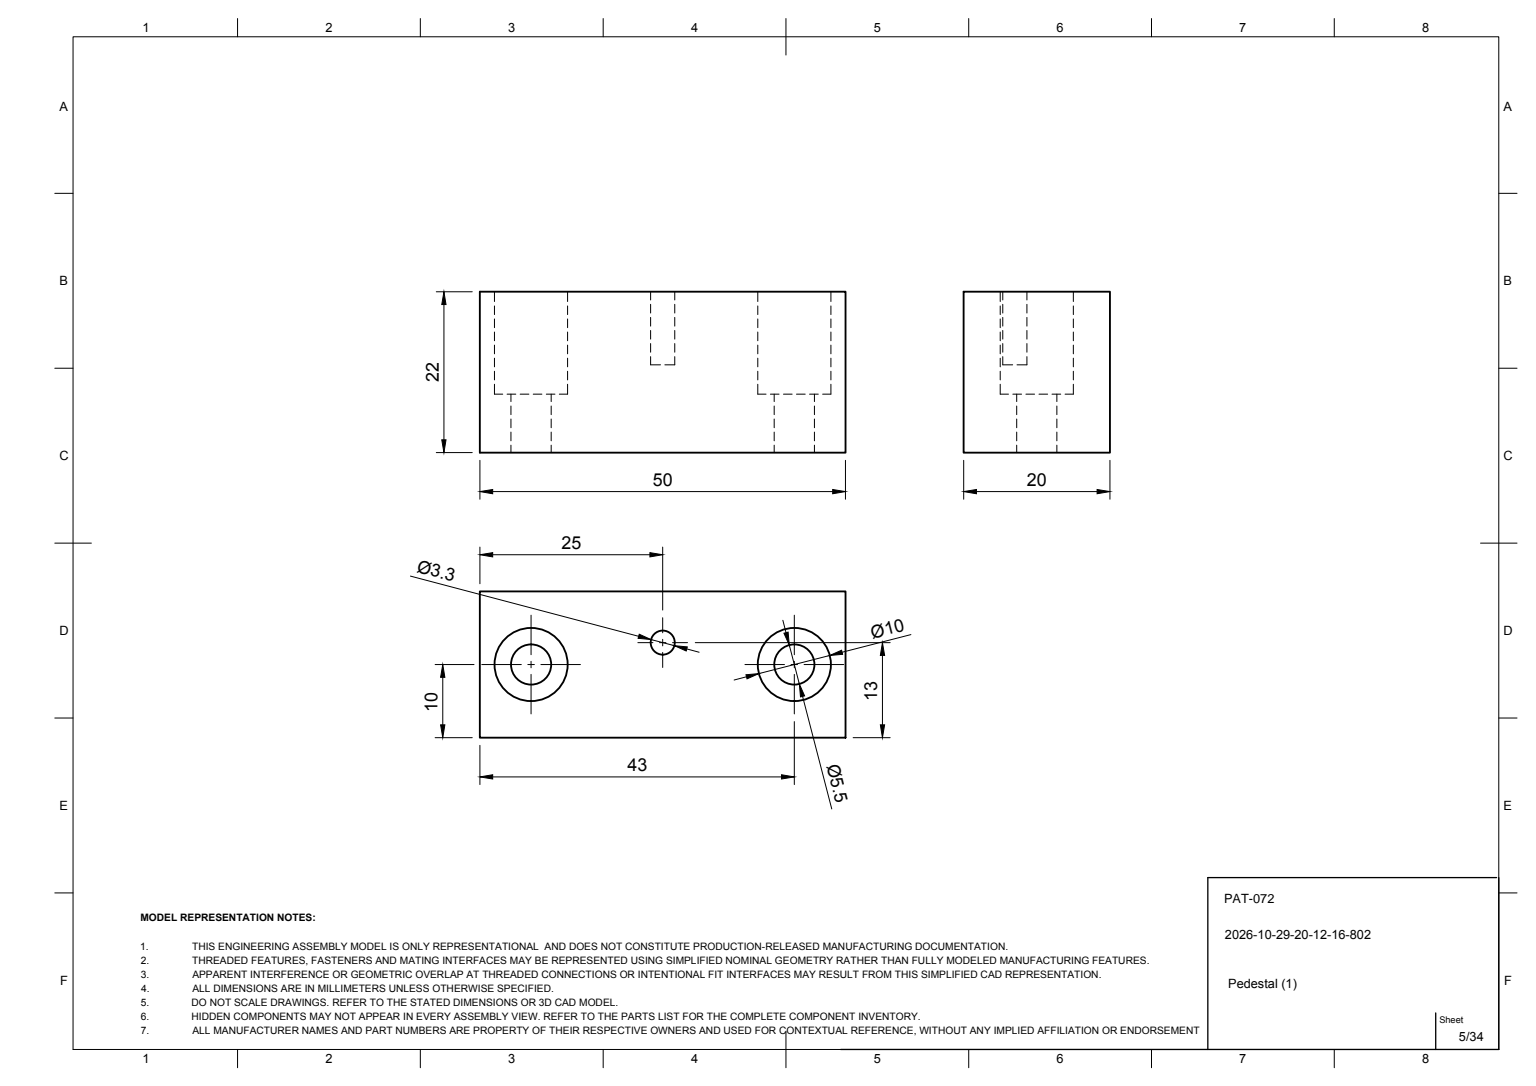
ISO-10303-21;
HEADER;
/* Generated by software containing ST-Developer
 * from STEP Tools, Inc. (www.steptools.com) 
 */

FILE_DESCRIPTION(
/* description */ ('PAT-072'),
/* implementation_level */ '2;1');

FILE_NAME(
/* name */ 'Pedestal (1).step',
/* time_stamp */ '2026-10-29T20:11:56-07:00',
/* author */ (''),
/* organization */ (''),
/* preprocessor_version */ 'ST-DEVELOPER v20.2',
/* originating_system */ 'Autodesk Translation Framework v15.17.0.0',
/* authorisation */ '');

FILE_SCHEMA (('AUTOMOTIVE_DESIGN { 1 0 10303 214 3 1 1 }'));
ENDSEC;

DATA;
#10=MECHANICAL_DESIGN_GEOMETRIC_PRESENTATION_REPRESENTATION('',(#334),#11432);
#262=SHAPE_REPRESENTATION_RELATIONSHIP('SRR','None',#11566,#298);
#298=ADVANCED_BREP_SHAPE_REPRESENTATION('',(#370),#11397);
#334=STYLED_ITEM('',(#11805),#370);
#370=MANIFOLD_SOLID_BREP('Body1',#6069);
#417=FACE_BOUND('',#1211,.T.);
#418=FACE_BOUND('',#1214,.T.);
#419=FACE_BOUND('',#1222,.T.);
#420=FACE_BOUND('',#1223,.T.);
#421=FACE_BOUND('',#1224,.T.);
#422=FACE_BOUND('',#1226,.T.);
#423=FACE_BOUND('',#1227,.T.);
#585=PLANE('',#6551);
#586=PLANE('',#6555);
#587=PLANE('',#6560);
#588=PLANE('',#6566);
#589=PLANE('',#6567);
#590=PLANE('',#6568);
#591=PLANE('',#6569);
#592=PLANE('',#6570);
#593=PLANE('',#6571);
#820=FACE_OUTER_BOUND('',#1207,.T.);
#821=FACE_OUTER_BOUND('',#1208,.T.);
#822=FACE_OUTER_BOUND('',#1209,.T.);
#823=FACE_OUTER_BOUND('',#1210,.T.);
#824=FACE_OUTER_BOUND('',#1212,.T.);
#825=FACE_OUTER_BOUND('',#1213,.T.);
#826=FACE_OUTER_BOUND('',#1215,.T.);
#827=FACE_OUTER_BOUND('',#1216,.T.);
#828=FACE_OUTER_BOUND('',#1217,.T.);
#829=FACE_OUTER_BOUND('',#1218,.T.);
#830=FACE_OUTER_BOUND('',#1219,.T.);
#831=FACE_OUTER_BOUND('',#1220,.T.);
#832=FACE_OUTER_BOUND('',#1221,.T.);
#833=FACE_OUTER_BOUND('',#1225,.T.);
#1207=EDGE_LOOP('',(#4170,#4171,#4172,#4173));
#1208=EDGE_LOOP('',(#4174));
#1209=EDGE_LOOP('',(#4175,#4176,#4177,#4178));
#1210=EDGE_LOOP('',(#4179));
#1211=EDGE_LOOP('',(#4180));
#1212=EDGE_LOOP('',(#4181,#4182,#4183,#4184));
#1213=EDGE_LOOP('',(#4185));
#1214=EDGE_LOOP('',(#4186));
#1215=EDGE_LOOP('',(#4187,#4188,#4189,#4190));
#1216=EDGE_LOOP('',(#4191,#4192,#4193,#4194));
#1217=EDGE_LOOP('',(#4195,#4196,#4197,#4198));
#1218=EDGE_LOOP('',(#4199,#4200,#4201,#4202));
#1219=EDGE_LOOP('',(#4203,#4204,#4205,#4206));
#1220=EDGE_LOOP('',(#4207,#4208,#4209,#4210));
#1221=EDGE_LOOP('',(#4211,#4212,#4213,#4214));
#1222=EDGE_LOOP('',(#4215));
#1223=EDGE_LOOP('',(#4216));
#1224=EDGE_LOOP('',(#4217));
#1225=EDGE_LOOP('',(#4218,#4219,#4220,#4221));
#1226=EDGE_LOOP('',(#4222));
#1227=EDGE_LOOP('',(#4223));
#1741=LINE('',#9309,#2160);
#1742=LINE('',#9316,#2161);
#1743=LINE('',#9325,#2162);
#1744=LINE('',#9333,#2163);
#1745=LINE('',#9337,#2164);
#1746=LINE('',#9341,#2165);
#1747=LINE('',#9343,#2166);
#1748=LINE('',#9345,#2167);
#1749=LINE('',#9346,#2168);
#1750=LINE('',#9349,#2169);
#1751=LINE('',#9351,#2170);
#1752=LINE('',#9352,#2171);
#1753=LINE('',#9355,#2172);
#1754=LINE('',#9357,#2173);
#1755=LINE('',#9358,#2174);
#1756=LINE('',#9360,#2175);
#1757=LINE('',#9361,#2176);
#2160=VECTOR('',#7388,0.165);
#2161=VECTOR('',#7397,0.5);
#2162=VECTOR('',#7408,0.5);
#2163=VECTOR('',#7419,0.275);
#2164=VECTOR('',#7424,0.275);
#2165=VECTOR('',#7427,1.);
#2166=VECTOR('',#7428,1.);
#2167=VECTOR('',#7429,1.);
#2168=VECTOR('',#7430,1.);
#2169=VECTOR('',#7433,1.);
#2170=VECTOR('',#7434,1.);
#2171=VECTOR('',#7435,1.);
#2172=VECTOR('',#7438,1.);
#2173=VECTOR('',#7439,1.);
#2174=VECTOR('',#7440,1.);
#2175=VECTOR('',#7443,1.);
#2176=VECTOR('',#7444,1.);
#2564=CIRCLE('',#6549,0.165);
#2565=CIRCLE('',#6550,0.165);
#2566=CIRCLE('',#6553,0.5);
#2567=CIRCLE('',#6554,0.5);
#2568=CIRCLE('',#6556,0.275);
#2569=CIRCLE('',#6558,0.5);
#2570=CIRCLE('',#6559,0.5);
#2571=CIRCLE('',#6561,0.275);
#2572=CIRCLE('',#6563,0.275);
#2573=CIRCLE('',#6565,0.275);
#2870=VERTEX_POINT('',#9306);
#2871=VERTEX_POINT('',#9308);
#2872=VERTEX_POINT('',#9313);
#2873=VERTEX_POINT('',#9315);
#2874=VERTEX_POINT('',#9319);
#2875=VERTEX_POINT('',#9322);
#2876=VERTEX_POINT('',#9324);
#2877=VERTEX_POINT('',#9328);
#2878=VERTEX_POINT('',#9331);
#2879=VERTEX_POINT('',#9335);
#2880=VERTEX_POINT('',#9339);
#2881=VERTEX_POINT('',#9340);
#2882=VERTEX_POINT('',#9342);
#2883=VERTEX_POINT('',#9344);
#2884=VERTEX_POINT('',#9348);
#2885=VERTEX_POINT('',#9350);
#2886=VERTEX_POINT('',#9354);
#2887=VERTEX_POINT('',#9356);
#3374=EDGE_CURVE('',#2870,#2870,#2564,.T.);
#3375=EDGE_CURVE('',#2870,#2871,#1741,.T.);
#3376=EDGE_CURVE('',#2871,#2871,#2565,.T.);
#3377=EDGE_CURVE('',#2872,#2872,#2566,.T.);
#3378=EDGE_CURVE('',#2872,#2873,#1742,.T.);
#3379=EDGE_CURVE('',#2873,#2873,#2567,.T.);
#3380=EDGE_CURVE('',#2874,#2874,#2568,.T.);
#3381=EDGE_CURVE('',#2875,#2875,#2569,.T.);
#3382=EDGE_CURVE('',#2875,#2876,#1743,.T.);
#3383=EDGE_CURVE('',#2876,#2876,#2570,.T.);
#3384=EDGE_CURVE('',#2877,#2877,#2571,.T.);
#3385=EDGE_CURVE('',#2878,#2878,#2572,.T.);
#3386=EDGE_CURVE('',#2878,#2874,#1744,.T.);
#3387=EDGE_CURVE('',#2879,#2879,#2573,.T.);
#3388=EDGE_CURVE('',#2879,#2877,#1745,.T.);
#3389=EDGE_CURVE('',#2880,#2881,#1746,.T.);
#3390=EDGE_CURVE('',#2881,#2882,#1747,.T.);
#3391=EDGE_CURVE('',#2883,#2882,#1748,.T.);
#3392=EDGE_CURVE('',#2880,#2883,#1749,.T.);
#3393=EDGE_CURVE('',#2884,#2880,#1750,.T.);
#3394=EDGE_CURVE('',#2885,#2883,#1751,.T.);
#3395=EDGE_CURVE('',#2884,#2885,#1752,.T.);
#3396=EDGE_CURVE('',#2886,#2884,#1753,.T.);
#3397=EDGE_CURVE('',#2887,#2885,#1754,.T.);
#3398=EDGE_CURVE('',#2886,#2887,#1755,.T.);
#3399=EDGE_CURVE('',#2881,#2886,#1756,.T.);
#3400=EDGE_CURVE('',#2882,#2887,#1757,.T.);
#4170=ORIENTED_EDGE('',*,*,#3374,.F.);
#4171=ORIENTED_EDGE('',*,*,#3375,.T.);
#4172=ORIENTED_EDGE('',*,*,#3376,.F.);
#4173=ORIENTED_EDGE('',*,*,#3375,.F.);
#4174=ORIENTED_EDGE('',*,*,#3374,.T.);
#4175=ORIENTED_EDGE('',*,*,#3377,.F.);
#4176=ORIENTED_EDGE('',*,*,#3378,.T.);
#4177=ORIENTED_EDGE('',*,*,#3379,.F.);
#4178=ORIENTED_EDGE('',*,*,#3378,.F.);
#4179=ORIENTED_EDGE('',*,*,#3377,.T.);
#4180=ORIENTED_EDGE('',*,*,#3380,.F.);
#4181=ORIENTED_EDGE('',*,*,#3381,.F.);
#4182=ORIENTED_EDGE('',*,*,#3382,.T.);
#4183=ORIENTED_EDGE('',*,*,#3383,.F.);
#4184=ORIENTED_EDGE('',*,*,#3382,.F.);
#4185=ORIENTED_EDGE('',*,*,#3381,.T.);
#4186=ORIENTED_EDGE('',*,*,#3384,.F.);
#4187=ORIENTED_EDGE('',*,*,#3385,.F.);
#4188=ORIENTED_EDGE('',*,*,#3386,.T.);
#4189=ORIENTED_EDGE('',*,*,#3380,.T.);
#4190=ORIENTED_EDGE('',*,*,#3386,.F.);
#4191=ORIENTED_EDGE('',*,*,#3387,.F.);
#4192=ORIENTED_EDGE('',*,*,#3388,.T.);
#4193=ORIENTED_EDGE('',*,*,#3384,.T.);
#4194=ORIENTED_EDGE('',*,*,#3388,.F.);
#4195=ORIENTED_EDGE('',*,*,#3389,.T.);
#4196=ORIENTED_EDGE('',*,*,#3390,.T.);
#4197=ORIENTED_EDGE('',*,*,#3391,.F.);
#4198=ORIENTED_EDGE('',*,*,#3392,.F.);
#4199=ORIENTED_EDGE('',*,*,#3393,.T.);
#4200=ORIENTED_EDGE('',*,*,#3392,.T.);
#4201=ORIENTED_EDGE('',*,*,#3394,.F.);
#4202=ORIENTED_EDGE('',*,*,#3395,.F.);
#4203=ORIENTED_EDGE('',*,*,#3396,.T.);
#4204=ORIENTED_EDGE('',*,*,#3395,.T.);
#4205=ORIENTED_EDGE('',*,*,#3397,.F.);
#4206=ORIENTED_EDGE('',*,*,#3398,.F.);
#4207=ORIENTED_EDGE('',*,*,#3399,.T.);
#4208=ORIENTED_EDGE('',*,*,#3398,.T.);
#4209=ORIENTED_EDGE('',*,*,#3400,.F.);
#4210=ORIENTED_EDGE('',*,*,#3390,.F.);
#4211=ORIENTED_EDGE('',*,*,#3400,.T.);
#4212=ORIENTED_EDGE('',*,*,#3397,.T.);
#4213=ORIENTED_EDGE('',*,*,#3394,.T.);
#4214=ORIENTED_EDGE('',*,*,#3391,.T.);
#4215=ORIENTED_EDGE('',*,*,#3376,.T.);
#4216=ORIENTED_EDGE('',*,*,#3379,.T.);
#4217=ORIENTED_EDGE('',*,*,#3383,.T.);
#4218=ORIENTED_EDGE('',*,*,#3399,.F.);
#4219=ORIENTED_EDGE('',*,*,#3389,.F.);
#4220=ORIENTED_EDGE('',*,*,#3393,.F.);
#4221=ORIENTED_EDGE('',*,*,#3396,.F.);
#4222=ORIENTED_EDGE('',*,*,#3385,.T.);
#4223=ORIENTED_EDGE('',*,*,#3387,.T.);
#5567=CYLINDRICAL_SURFACE('',#6548,0.165);
#5568=CYLINDRICAL_SURFACE('',#6552,0.5);
#5569=CYLINDRICAL_SURFACE('',#6557,0.5);
#5570=CYLINDRICAL_SURFACE('',#6562,0.275);
#5571=CYLINDRICAL_SURFACE('',#6564,0.275);
#5719=ADVANCED_FACE('',(#820),#5567,.F.);
#5720=ADVANCED_FACE('',(#821),#585,.T.);
#5721=ADVANCED_FACE('',(#822),#5568,.F.);
#5722=ADVANCED_FACE('',(#823,#417),#586,.T.);
#5723=ADVANCED_FACE('',(#824),#5569,.F.);
#5724=ADVANCED_FACE('',(#825,#418),#587,.T.);
#5725=ADVANCED_FACE('',(#826),#5570,.F.);
#5726=ADVANCED_FACE('',(#827),#5571,.F.);
#5727=ADVANCED_FACE('',(#828),#588,.T.);
#5728=ADVANCED_FACE('',(#829),#589,.T.);
#5729=ADVANCED_FACE('',(#830),#590,.T.);
#5730=ADVANCED_FACE('',(#831),#591,.T.);
#5731=ADVANCED_FACE('',(#832,#419,#420,#421),#592,.T.);
#5732=ADVANCED_FACE('',(#833,#422,#423),#593,.F.);
#6069=CLOSED_SHELL('',(#5719,#5720,#5721,#5722,#5723,#5724,#5725,#5726,
#5727,#5728,#5729,#5730,#5731,#5732));
#6547=AXIS2_PLACEMENT_3D('',#9304,#7382,#7383);
#6548=AXIS2_PLACEMENT_3D('',#9305,#7384,#7385);
#6549=AXIS2_PLACEMENT_3D('',#9307,#7386,#7387);
#6550=AXIS2_PLACEMENT_3D('',#9310,#7389,#7390);
#6551=AXIS2_PLACEMENT_3D('',#9311,#7391,#7392);
#6552=AXIS2_PLACEMENT_3D('',#9312,#7393,#7394);
#6553=AXIS2_PLACEMENT_3D('',#9314,#7395,#7396);
#6554=AXIS2_PLACEMENT_3D('',#9317,#7398,#7399);
#6555=AXIS2_PLACEMENT_3D('',#9318,#7400,#7401);
#6556=AXIS2_PLACEMENT_3D('',#9320,#7402,#7403);
#6557=AXIS2_PLACEMENT_3D('',#9321,#7404,#7405);
#6558=AXIS2_PLACEMENT_3D('',#9323,#7406,#7407);
#6559=AXIS2_PLACEMENT_3D('',#9326,#7409,#7410);
#6560=AXIS2_PLACEMENT_3D('',#9327,#7411,#7412);
#6561=AXIS2_PLACEMENT_3D('',#9329,#7413,#7414);
#6562=AXIS2_PLACEMENT_3D('',#9330,#7415,#7416);
#6563=AXIS2_PLACEMENT_3D('',#9332,#7417,#7418);
#6564=AXIS2_PLACEMENT_3D('',#9334,#7420,#7421);
#6565=AXIS2_PLACEMENT_3D('',#9336,#7422,#7423);
#6566=AXIS2_PLACEMENT_3D('',#9338,#7425,#7426);
#6567=AXIS2_PLACEMENT_3D('',#9347,#7431,#7432);
#6568=AXIS2_PLACEMENT_3D('',#9353,#7436,#7437);
#6569=AXIS2_PLACEMENT_3D('',#9359,#7441,#7442);
#6570=AXIS2_PLACEMENT_3D('',#9362,#7445,#7446);
#6571=AXIS2_PLACEMENT_3D('',#9363,#7447,#7448);
#7382=DIRECTION('axis',(0.,0.,1.));
#7383=DIRECTION('refdir',(1.,0.,0.));
#7384=DIRECTION('center_axis',(0.,0.,1.));
#7385=DIRECTION('ref_axis',(1.,0.,0.));
#7386=DIRECTION('center_axis',(0.,0.,1.));
#7387=DIRECTION('ref_axis',(1.,0.,0.));
#7388=DIRECTION('',(0.,0.,1.));
#7389=DIRECTION('center_axis',(0.,0.,-1.));
#7390=DIRECTION('ref_axis',(1.,0.,0.));
#7391=DIRECTION('center_axis',(0.,0.,1.));
#7392=DIRECTION('ref_axis',(1.,0.,0.));
#7393=DIRECTION('center_axis',(0.,0.,1.));
#7394=DIRECTION('ref_axis',(1.,0.,0.));
#7395=DIRECTION('center_axis',(0.,0.,1.));
#7396=DIRECTION('ref_axis',(1.,0.,0.));
#7397=DIRECTION('',(0.,0.,1.));
#7398=DIRECTION('center_axis',(0.,0.,-1.));
#7399=DIRECTION('ref_axis',(1.,0.,0.));
#7400=DIRECTION('center_axis',(0.,0.,1.));
#7401=DIRECTION('ref_axis',(1.,0.,0.));
#7402=DIRECTION('center_axis',(0.,0.,1.));
#7403=DIRECTION('ref_axis',(1.,0.,0.));
#7404=DIRECTION('center_axis',(0.,0.,1.));
#7405=DIRECTION('ref_axis',(1.,0.,0.));
#7406=DIRECTION('center_axis',(0.,0.,1.));
#7407=DIRECTION('ref_axis',(1.,0.,0.));
#7408=DIRECTION('',(0.,0.,1.));
#7409=DIRECTION('center_axis',(0.,0.,-1.));
#7410=DIRECTION('ref_axis',(1.,0.,0.));
#7411=DIRECTION('center_axis',(0.,0.,1.));
#7412=DIRECTION('ref_axis',(1.,0.,0.));
#7413=DIRECTION('center_axis',(0.,0.,1.));
#7414=DIRECTION('ref_axis',(1.,0.,0.));
#7415=DIRECTION('center_axis',(0.,0.,1.));
#7416=DIRECTION('ref_axis',(1.,0.,0.));
#7417=DIRECTION('center_axis',(0.,0.,1.));
#7418=DIRECTION('ref_axis',(1.,0.,0.));
#7419=DIRECTION('',(0.,0.,1.));
#7420=DIRECTION('center_axis',(0.,0.,1.));
#7421=DIRECTION('ref_axis',(1.,0.,0.));
#7422=DIRECTION('center_axis',(0.,0.,1.));
#7423=DIRECTION('ref_axis',(1.,0.,0.));
#7424=DIRECTION('',(0.,0.,1.));
#7425=DIRECTION('center_axis',(0.,1.,0.));
#7426=DIRECTION('ref_axis',(-1.,0.,0.));
#7427=DIRECTION('',(-1.,0.,0.));
#7428=DIRECTION('',(0.,0.,1.));
#7429=DIRECTION('',(-1.,0.,0.));
#7430=DIRECTION('',(0.,0.,1.));
#7431=DIRECTION('center_axis',(1.,0.,0.));
#7432=DIRECTION('ref_axis',(0.,1.,0.));
#7433=DIRECTION('',(0.,1.,0.));
#7434=DIRECTION('',(0.,1.,0.));
#7435=DIRECTION('',(0.,0.,1.));
#7436=DIRECTION('center_axis',(0.,-1.,0.));
#7437=DIRECTION('ref_axis',(1.,0.,0.));
#7438=DIRECTION('',(1.,0.,0.));
#7439=DIRECTION('',(1.,0.,0.));
#7440=DIRECTION('',(0.,0.,1.));
#7441=DIRECTION('center_axis',(-1.,0.,0.));
#7442=DIRECTION('ref_axis',(0.,-1.,0.));
#7443=DIRECTION('',(0.,-1.,0.));
#7444=DIRECTION('',(0.,-1.,0.));
#7445=DIRECTION('center_axis',(0.,0.,1.));
#7446=DIRECTION('ref_axis',(1.,0.,0.));
#7447=DIRECTION('center_axis',(0.,0.,1.));
#7448=DIRECTION('ref_axis',(1.,0.,0.));
#9304=CARTESIAN_POINT('',(0.,0.,0.));
#9305=CARTESIAN_POINT('Origin',(4.8,0.,2.));
#9306=CARTESIAN_POINT('',(4.635,-2.02066721859313E-17,2.));
#9307=CARTESIAN_POINT('Origin',(4.8,0.,2.));
#9308=CARTESIAN_POINT('',(4.635,2.02066721859313E-17,3.));
#9309=CARTESIAN_POINT('',(4.635,-2.02066721859313E-17,2.));
#9310=CARTESIAN_POINT('Origin',(4.8,0.,3.));
#9311=CARTESIAN_POINT('Origin',(4.8,0.,2.));
#9312=CARTESIAN_POINT('Origin',(4.5,-1.8,1.6));
#9313=CARTESIAN_POINT('',(4.,-1.8,1.6));
#9314=CARTESIAN_POINT('Origin',(4.5,-1.8,1.6));
#9315=CARTESIAN_POINT('',(4.,-1.8,3.));
#9316=CARTESIAN_POINT('',(4.,-1.8,1.6));
#9317=CARTESIAN_POINT('Origin',(4.5,-1.8,3.));
#9318=CARTESIAN_POINT('Origin',(4.5,-1.8,1.6));
#9319=CARTESIAN_POINT('',(4.225,-1.8,1.6));
#9320=CARTESIAN_POINT('Origin',(4.5,-1.8,1.6));
#9321=CARTESIAN_POINT('Origin',(4.5,1.8,1.6));
#9322=CARTESIAN_POINT('',(4.,1.8,1.6));
#9323=CARTESIAN_POINT('Origin',(4.5,1.8,1.6));
#9324=CARTESIAN_POINT('',(4.,1.8,3.));
#9325=CARTESIAN_POINT('',(4.,1.8,1.6));
#9326=CARTESIAN_POINT('Origin',(4.5,1.8,3.));
#9327=CARTESIAN_POINT('Origin',(4.5,1.8,1.6));
#9328=CARTESIAN_POINT('',(4.225,1.8,1.6));
#9329=CARTESIAN_POINT('Origin',(4.5,1.8,1.6));
#9330=CARTESIAN_POINT('Origin',(4.5,-1.8,0.7));
#9331=CARTESIAN_POINT('',(4.225,-1.8,0.8));
#9332=CARTESIAN_POINT('Origin',(4.5,-1.8,0.8));
#9333=CARTESIAN_POINT('',(4.225,-1.8,0.7));
#9334=CARTESIAN_POINT('Origin',(4.5,1.8,0.7));
#9335=CARTESIAN_POINT('',(4.225,1.8,0.8));
#9336=CARTESIAN_POINT('Origin',(4.5,1.8,0.8));
#9337=CARTESIAN_POINT('',(4.225,1.8,0.7));
#9338=CARTESIAN_POINT('Origin',(5.5,2.5,0.8));
#9339=CARTESIAN_POINT('',(5.5,2.5,0.8));
#9340=CARTESIAN_POINT('',(3.5,2.5,0.8));
#9341=CARTESIAN_POINT('',(5.5,2.5,0.8));
#9342=CARTESIAN_POINT('',(3.5,2.5,3.));
#9343=CARTESIAN_POINT('',(3.5,2.5,0.8));
#9344=CARTESIAN_POINT('',(5.5,2.5,3.));
#9345=CARTESIAN_POINT('',(5.5,2.5,3.));
#9346=CARTESIAN_POINT('',(5.5,2.5,0.8));
#9347=CARTESIAN_POINT('Origin',(5.5,-2.5,0.8));
#9348=CARTESIAN_POINT('',(5.5,-2.5,0.8));
#9349=CARTESIAN_POINT('',(5.5,-2.5,0.8));
#9350=CARTESIAN_POINT('',(5.5,-2.5,3.));
#9351=CARTESIAN_POINT('',(5.5,-2.5,3.));
#9352=CARTESIAN_POINT('',(5.5,-2.5,0.8));
#9353=CARTESIAN_POINT('Origin',(3.5,-2.5,0.8));
#9354=CARTESIAN_POINT('',(3.5,-2.5,0.8));
#9355=CARTESIAN_POINT('',(3.5,-2.5,0.8));
#9356=CARTESIAN_POINT('',(3.5,-2.5,3.));
#9357=CARTESIAN_POINT('',(3.5,-2.5,3.));
#9358=CARTESIAN_POINT('',(3.5,-2.5,0.8));
#9359=CARTESIAN_POINT('Origin',(3.5,2.5,0.8));
#9360=CARTESIAN_POINT('',(3.5,2.5,0.8));
#9361=CARTESIAN_POINT('',(3.5,2.5,3.));
#9362=CARTESIAN_POINT('Origin',(4.5,0.,3.));
#9363=CARTESIAN_POINT('Origin',(4.5,0.,0.8));
#11358=UNCERTAINTY_MEASURE_WITH_UNIT(LENGTH_MEASURE(0.001),#11433,
'DISTANCE_ACCURACY_VALUE',
'Maximum model space distance between geometric entities at asserted c
onnectivities');
#11393=UNCERTAINTY_MEASURE_WITH_UNIT(LENGTH_MEASURE(0.001),#11433,
'DISTANCE_ACCURACY_VALUE',
'Maximum model space distance between geometric entities at asserted c
onnectivities');
#11397=(
GEOMETRIC_REPRESENTATION_CONTEXT(3)
GLOBAL_UNCERTAINTY_ASSIGNED_CONTEXT((#11358))
GLOBAL_UNIT_ASSIGNED_CONTEXT((#11433,#11435,#11436))
REPRESENTATION_CONTEXT('','3D')
);
#11432=(
GEOMETRIC_REPRESENTATION_CONTEXT(3)
GLOBAL_UNCERTAINTY_ASSIGNED_CONTEXT((#11393))
GLOBAL_UNIT_ASSIGNED_CONTEXT((#11433,#11435,#11436))
REPRESENTATION_CONTEXT('','3D')
);
#11433=(
LENGTH_UNIT()
NAMED_UNIT(*)
SI_UNIT(.CENTI.,.METRE.)
);
#11435=(
NAMED_UNIT(*)
PLANE_ANGLE_UNIT()
SI_UNIT($,.RADIAN.)
);
#11436=(
NAMED_UNIT(*)
SI_UNIT($,.STERADIAN.)
SOLID_ANGLE_UNIT()
);
#11440=SHAPE_DEFINITION_REPRESENTATION(#11478,#11566);
#11478=PRODUCT_DEFINITION_SHAPE('',$,#11605);
#11566=SHAPE_REPRESENTATION('',(#6547),#11397);
#11601=PRODUCT_DEFINITION_CONTEXT('part definition',#11717,'design');
#11605=PRODUCT_DEFINITION('Pedestal (1)','Pedestal (1)',#11643,
#11601);
#11643=PRODUCT_DEFINITION_FORMATION('',$,#11722);
#11717=APPLICATION_CONTEXT(
'Core Data for Automotive Mechanical Design Process');
#11718=PRODUCT_CONTEXT('part definition',#11717,'mechanical');
#11722=PRODUCT('Pedestal (1)','Pedestal (1)','Pedestal (1)',(#11718));
#11799=COLOUR_RGB('Light Blue',0.38,0.62,0.78);
#11800=FILL_AREA_STYLE_COLOUR('',#11799);
#11801=FILL_AREA_STYLE('',(#11800));
#11802=SURFACE_STYLE_FILL_AREA(#11801);
#11803=SURFACE_SIDE_STYLE('',(#11802));
#11804=SURFACE_STYLE_USAGE(.BOTH.,#11803);
#11805=PRESENTATION_STYLE_ASSIGNMENT((#11804));
ENDSEC;
END-ISO-10303-21;
